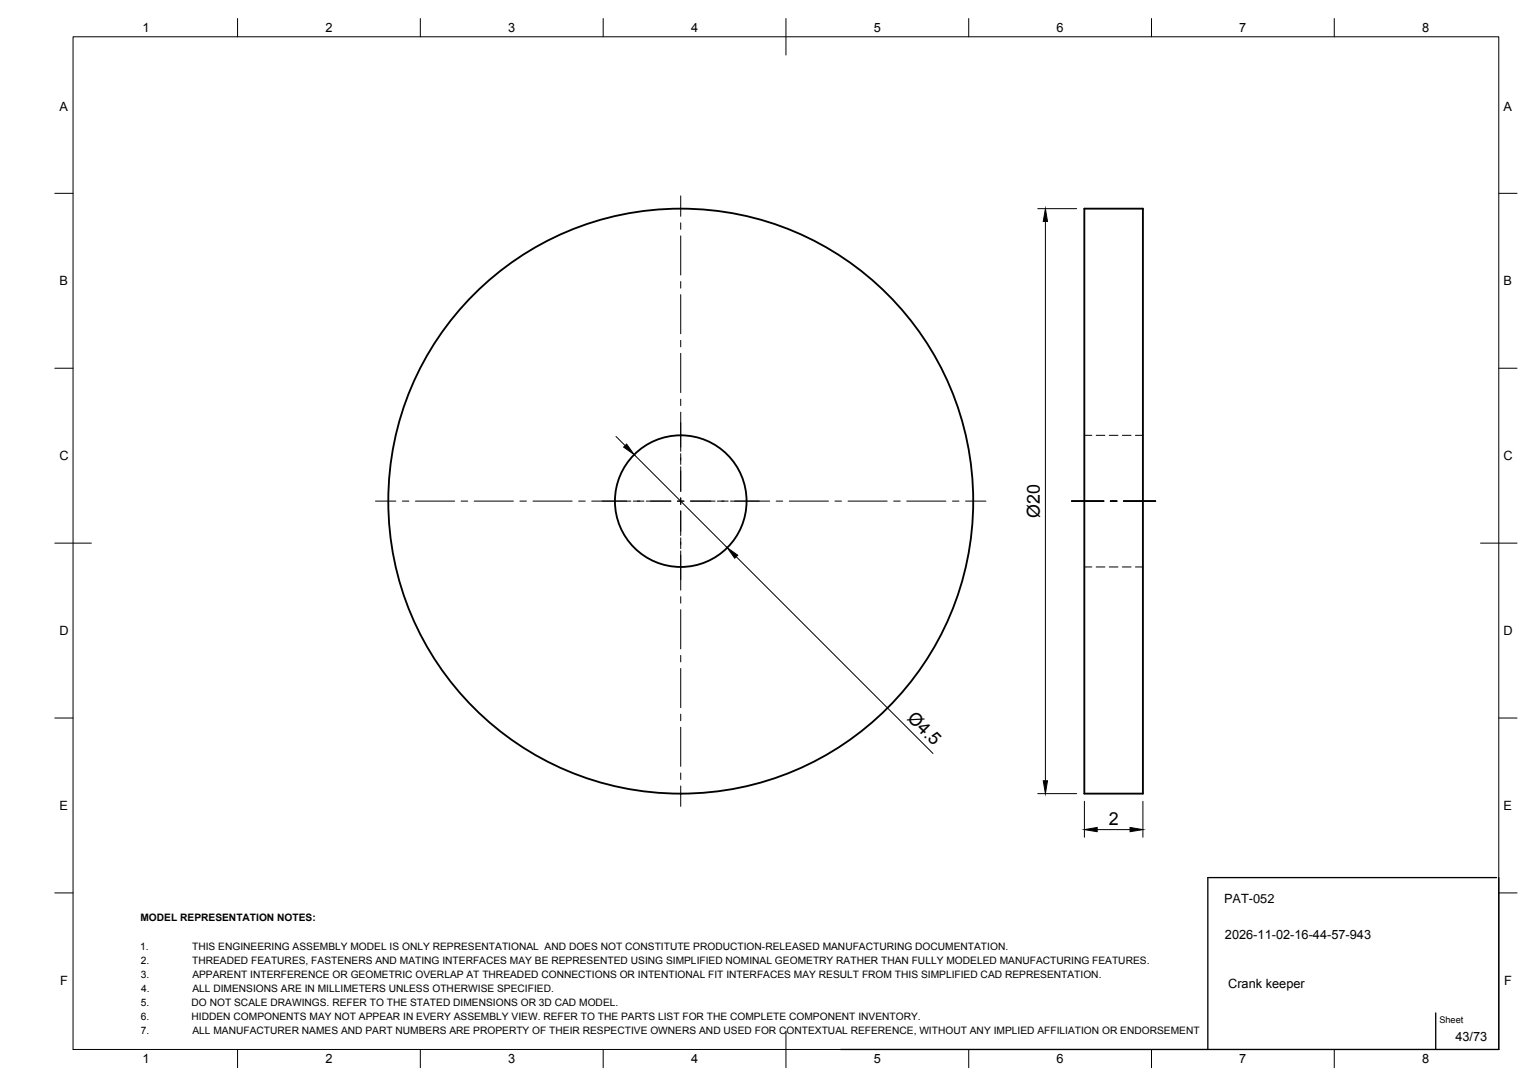
ISO-10303-21;
HEADER;
/* Generated by software containing ST-Developer
 * from STEP Tools, Inc. (www.steptools.com) 
 */

FILE_DESCRIPTION(
/* description */ ('Hand-crank gear train demonstrator'),
/* implementation_level */ '2;1');

FILE_NAME(
/* name */ 'Crank keeper.step',
/* time_stamp */ '2026-10-28T03:22:13-07:00',
/* author */ (''),
/* organization */ (''),
/* preprocessor_version */ 'ST-DEVELOPER v20.2',
/* originating_system */ 'Autodesk Translation Framework v15.17.0.0',
/* authorisation */ '');

FILE_SCHEMA (('AUTOMOTIVE_DESIGN { 1 0 10303 214 3 1 1 }'));
ENDSEC;

DATA;
#10=MECHANICAL_DESIGN_GEOMETRIC_PRESENTATION_REPRESENTATION('',(#1239),#62758);
#1096=SHAPE_REPRESENTATION_RELATIONSHIP('SRR','None',#63071,#1160);
#1160=ADVANCED_BREP_SHAPE_REPRESENTATION('',(#1315),#62725);
#1239=STYLED_ITEM('',(#63448),#1315);
#1315=MANIFOLD_SOLID_BREP('Body1',#16422);
#1564=FACE_BOUND('',#3763,.T.);
#1565=FACE_BOUND('',#3765,.T.);
#1919=PLANE('',#18087);
#1920=PLANE('',#18088);
#2602=FACE_OUTER_BOUND('',#3760,.T.);
#2603=FACE_OUTER_BOUND('',#3761,.T.);
#2604=FACE_OUTER_BOUND('',#3762,.T.);
#2605=FACE_OUTER_BOUND('',#3764,.T.);
#3760=EDGE_LOOP('',(#12921,#12922,#12923,#12924));
#3761=EDGE_LOOP('',(#12925,#12926,#12927,#12928));
#3762=EDGE_LOOP('',(#12929));
#3763=EDGE_LOOP('',(#12930));
#3764=EDGE_LOOP('',(#12931));
#3765=EDGE_LOOP('',(#12932));
#4900=LINE('',#26280,#6032);
#4901=LINE('',#26286,#6033);
#6032=VECTOR('',#21295,0.225);
#6033=VECTOR('',#21302,1.);
#6943=CIRCLE('',#18082,0.225);
#6944=CIRCLE('',#18083,0.225);
#6945=CIRCLE('',#18085,1.);
#6946=CIRCLE('',#18086,1.);
#7922=VERTEX_POINT('',#26277);
#7923=VERTEX_POINT('',#26279);
#7924=VERTEX_POINT('',#26283);
#7925=VERTEX_POINT('',#26285);
#9712=EDGE_CURVE('',#7922,#7922,#6943,.T.);
#9713=EDGE_CURVE('',#7922,#7923,#4900,.T.);
#9714=EDGE_CURVE('',#7923,#7923,#6944,.T.);
#9715=EDGE_CURVE('',#7924,#7924,#6945,.T.);
#9716=EDGE_CURVE('',#7924,#7925,#4901,.T.);
#9717=EDGE_CURVE('',#7925,#7925,#6946,.T.);
#12921=ORIENTED_EDGE('',*,*,#9712,.F.);
#12922=ORIENTED_EDGE('',*,*,#9713,.T.);
#12923=ORIENTED_EDGE('',*,*,#9714,.T.);
#12924=ORIENTED_EDGE('',*,*,#9713,.F.);
#12925=ORIENTED_EDGE('',*,*,#9715,.F.);
#12926=ORIENTED_EDGE('',*,*,#9716,.T.);
#12927=ORIENTED_EDGE('',*,*,#9717,.T.);
#12928=ORIENTED_EDGE('',*,*,#9716,.F.);
#12929=ORIENTED_EDGE('',*,*,#9715,.T.);
#12930=ORIENTED_EDGE('',*,*,#9712,.T.);
#12931=ORIENTED_EDGE('',*,*,#9717,.F.);
#12932=ORIENTED_EDGE('',*,*,#9714,.F.);
#15309=CYLINDRICAL_SURFACE('',#18081,0.225);
#15310=CYLINDRICAL_SURFACE('',#18084,1.);
#15912=ADVANCED_FACE('',(#2602),#15309,.F.);
#15913=ADVANCED_FACE('',(#2603),#15310,.T.);
#15914=ADVANCED_FACE('',(#2604,#1564),#1919,.T.);
#15915=ADVANCED_FACE('',(#2605,#1565),#1920,.F.);
#16422=CLOSED_SHELL('',(#15912,#15913,#15914,#15915));
#18080=AXIS2_PLACEMENT_3D('',#26275,#21289,#21290);
#18081=AXIS2_PLACEMENT_3D('',#26276,#21291,#21292);
#18082=AXIS2_PLACEMENT_3D('',#26278,#21293,#21294);
#18083=AXIS2_PLACEMENT_3D('',#26281,#21296,#21297);
#18084=AXIS2_PLACEMENT_3D('',#26282,#21298,#21299);
#18085=AXIS2_PLACEMENT_3D('',#26284,#21300,#21301);
#18086=AXIS2_PLACEMENT_3D('',#26287,#21303,#21304);
#18087=AXIS2_PLACEMENT_3D('',#26288,#21305,#21306);
#18088=AXIS2_PLACEMENT_3D('',#26289,#21307,#21308);
#21289=DIRECTION('axis',(0.,0.,1.));
#21290=DIRECTION('refdir',(1.,0.,0.));
#21291=DIRECTION('center_axis',(0.,1.,0.));
#21292=DIRECTION('ref_axis',(1.,0.,0.));
#21293=DIRECTION('center_axis',(0.,-1.,0.));
#21294=DIRECTION('ref_axis',(1.,0.,0.));
#21295=DIRECTION('',(0.,-1.,0.));
#21296=DIRECTION('center_axis',(0.,-1.,0.));
#21297=DIRECTION('ref_axis',(1.,0.,0.));
#21298=DIRECTION('center_axis',(0.,1.,0.));
#21299=DIRECTION('ref_axis',(1.,0.,0.));
#21300=DIRECTION('center_axis',(0.,1.,0.));
#21301=DIRECTION('ref_axis',(1.,0.,0.));
#21302=DIRECTION('',(0.,-1.,0.));
#21303=DIRECTION('center_axis',(0.,1.,0.));
#21304=DIRECTION('ref_axis',(1.,0.,0.));
#21305=DIRECTION('center_axis',(0.,1.,0.));
#21306=DIRECTION('ref_axis',(1.,0.,0.));
#21307=DIRECTION('center_axis',(0.,1.,0.));
#21308=DIRECTION('ref_axis',(1.,0.,0.));
#26275=CARTESIAN_POINT('',(0.,0.,0.));
#26276=CARTESIAN_POINT('Origin',(0.,6.,9.));
#26277=CARTESIAN_POINT('',(-0.225,6.2,9.));
#26278=CARTESIAN_POINT('Origin',(0.,6.2,9.));
#26279=CARTESIAN_POINT('',(-0.225,6.,9.));
#26280=CARTESIAN_POINT('',(-0.225,6.,9.));
#26281=CARTESIAN_POINT('Origin',(0.,6.,9.));
#26282=CARTESIAN_POINT('Origin',(0.,6.,9.));
#26283=CARTESIAN_POINT('',(-1.,6.2,9.));
#26284=CARTESIAN_POINT('Origin',(0.,6.2,9.));
#26285=CARTESIAN_POINT('',(-1.,6.,9.));
#26286=CARTESIAN_POINT('',(-1.,6.,9.));
#26287=CARTESIAN_POINT('Origin',(0.,6.,9.));
#26288=CARTESIAN_POINT('Origin',(0.,6.2,9.));
#26289=CARTESIAN_POINT('Origin',(0.,6.,9.));
#62651=UNCERTAINTY_MEASURE_WITH_UNIT(LENGTH_MEASURE(0.001),#62759,
'DISTANCE_ACCURACY_VALUE',
'Maximum model space distance between geometric entities at asserted c
onnectivities');
#62684=UNCERTAINTY_MEASURE_WITH_UNIT(LENGTH_MEASURE(0.001),#62759,
'DISTANCE_ACCURACY_VALUE',
'Maximum model space distance between geometric entities at asserted c
onnectivities');
#62725=(
GEOMETRIC_REPRESENTATION_CONTEXT(3)
GLOBAL_UNCERTAINTY_ASSIGNED_CONTEXT((#62651))
GLOBAL_UNIT_ASSIGNED_CONTEXT((#62759,#62761,#62762))
REPRESENTATION_CONTEXT('','3D')
);
#62758=(
GEOMETRIC_REPRESENTATION_CONTEXT(3)
GLOBAL_UNCERTAINTY_ASSIGNED_CONTEXT((#62684))
GLOBAL_UNIT_ASSIGNED_CONTEXT((#62759,#62761,#62762))
REPRESENTATION_CONTEXT('','3D')
);
#62759=(
LENGTH_UNIT()
NAMED_UNIT(*)
SI_UNIT(.CENTI.,.METRE.)
);
#62761=(
NAMED_UNIT(*)
PLANE_ANGLE_UNIT()
SI_UNIT($,.RADIAN.)
);
#62762=(
NAMED_UNIT(*)
SI_UNIT($,.STERADIAN.)
SOLID_ANGLE_UNIT()
);
#62803=SHAPE_DEFINITION_REPRESENTATION(#62886,#63071);
#62886=PRODUCT_DEFINITION_SHAPE('',$,#63145);
#63071=SHAPE_REPRESENTATION('',(#18080),#62725);
#63104=PRODUCT_DEFINITION_CONTEXT('part definition',#63325,'design');
#63145=PRODUCT_DEFINITION('Crank keeper','Crank keeper',#63218,#63104);
#63218=PRODUCT_DEFINITION_FORMATION('',$,#63367);
#63325=APPLICATION_CONTEXT(
'Core Data for Automotive Mechanical Design Process');
#63326=PRODUCT_CONTEXT('part definition',#63325,'mechanical');
#63367=PRODUCT('Crank keeper','Crank keeper','Crank keeper',(#63326));
#63442=COLOUR_RGB('Light Blue',0.38,0.62,0.78);
#63443=FILL_AREA_STYLE_COLOUR('',#63442);
#63444=FILL_AREA_STYLE('',(#63443));
#63445=SURFACE_STYLE_FILL_AREA(#63444);
#63446=SURFACE_SIDE_STYLE('',(#63445));
#63447=SURFACE_STYLE_USAGE(.BOTH.,#63446);
#63448=PRESENTATION_STYLE_ASSIGNMENT((#63447));
ENDSEC;
END-ISO-10303-21;
